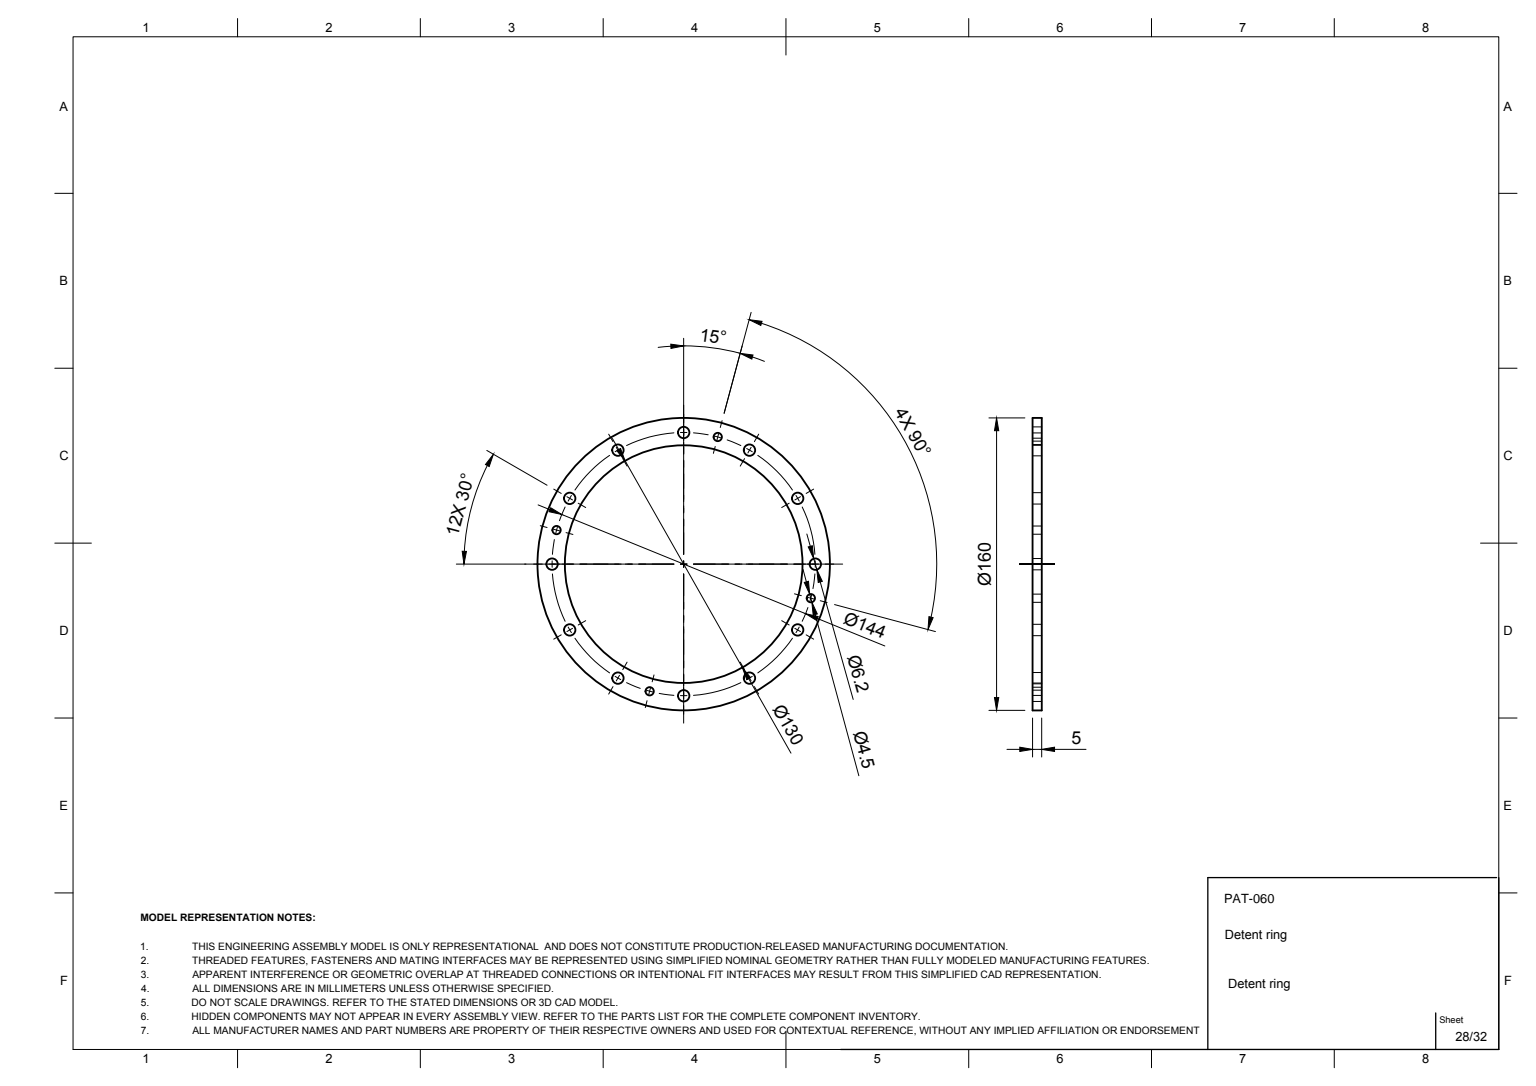
ISO-10303-21;
HEADER;
/* Generated by software containing ST-Developer
 * from STEP Tools, Inc. (www.steptools.com) 
 */

FILE_DESCRIPTION(
/* description */ ('Indexing fixture plate with plunger'),
/* implementation_level */ '2;1');

FILE_NAME(
/* name */ 'Detent ring.step',
/* time_stamp */ '2026-10-28T03:23:41-07:00',
/* author */ (''),
/* organization */ (''),
/* preprocessor_version */ 'ST-DEVELOPER v20.2',
/* originating_system */ 'Autodesk Translation Framework v15.17.0.0',
/* authorisation */ '');

FILE_SCHEMA (('AUTOMOTIVE_DESIGN { 1 0 10303 214 3 1 1 }'));
ENDSEC;

DATA;
#10=MECHANICAL_DESIGN_GEOMETRIC_PRESENTATION_REPRESENTATION('',(#348),#10020);
#285=SHAPE_REPRESENTATION_RELATIONSHIP('SRR','None',#10161,#312);
#312=ADVANCED_BREP_SHAPE_REPRESENTATION('',(#383),#10014);
#348=STYLED_ITEM('',(#10354),#383);
#383=MANIFOLD_SOLID_BREP('Body1',#4603);
#495=FACE_BOUND('',#1306,.T.);
#496=FACE_BOUND('',#1307,.T.);
#497=FACE_BOUND('',#1308,.T.);
#498=FACE_BOUND('',#1309,.T.);
#499=FACE_BOUND('',#1310,.T.);
#500=FACE_BOUND('',#1311,.T.);
#501=FACE_BOUND('',#1312,.T.);
#502=FACE_BOUND('',#1313,.T.);
#503=FACE_BOUND('',#1314,.T.);
#504=FACE_BOUND('',#1315,.T.);
#505=FACE_BOUND('',#1316,.T.);
#506=FACE_BOUND('',#1317,.T.);
#507=FACE_BOUND('',#1318,.T.);
#508=FACE_BOUND('',#1319,.T.);
#509=FACE_BOUND('',#1320,.T.);
#510=FACE_BOUND('',#1321,.T.);
#511=FACE_BOUND('',#1322,.T.);
#512=FACE_BOUND('',#1324,.T.);
#513=FACE_BOUND('',#1325,.T.);
#514=FACE_BOUND('',#1326,.T.);
#515=FACE_BOUND('',#1327,.T.);
#516=FACE_BOUND('',#1328,.T.);
#517=FACE_BOUND('',#1329,.T.);
#518=FACE_BOUND('',#1330,.T.);
#519=FACE_BOUND('',#1331,.T.);
#520=FACE_BOUND('',#1332,.T.);
#521=FACE_BOUND('',#1333,.T.);
#522=FACE_BOUND('',#1334,.T.);
#523=FACE_BOUND('',#1335,.T.);
#524=FACE_BOUND('',#1336,.T.);
#525=FACE_BOUND('',#1337,.T.);
#526=FACE_BOUND('',#1338,.T.);
#527=FACE_BOUND('',#1339,.T.);
#528=FACE_BOUND('',#1340,.T.);
#640=PLANE('',#5458);
#641=PLANE('',#5459);
#893=FACE_OUTER_BOUND('',#1287,.T.);
#894=FACE_OUTER_BOUND('',#1288,.T.);
#895=FACE_OUTER_BOUND('',#1289,.T.);
#896=FACE_OUTER_BOUND('',#1290,.T.);
#897=FACE_OUTER_BOUND('',#1291,.T.);
#898=FACE_OUTER_BOUND('',#1292,.T.);
#899=FACE_OUTER_BOUND('',#1293,.T.);
#900=FACE_OUTER_BOUND('',#1294,.T.);
#901=FACE_OUTER_BOUND('',#1295,.T.);
#902=FACE_OUTER_BOUND('',#1296,.T.);
#903=FACE_OUTER_BOUND('',#1297,.T.);
#904=FACE_OUTER_BOUND('',#1298,.T.);
#905=FACE_OUTER_BOUND('',#1299,.T.);
#906=FACE_OUTER_BOUND('',#1300,.T.);
#907=FACE_OUTER_BOUND('',#1301,.T.);
#908=FACE_OUTER_BOUND('',#1302,.T.);
#909=FACE_OUTER_BOUND('',#1303,.T.);
#910=FACE_OUTER_BOUND('',#1304,.T.);
#911=FACE_OUTER_BOUND('',#1305,.T.);
#912=FACE_OUTER_BOUND('',#1323,.T.);
#1287=EDGE_LOOP('',(#3895,#3896,#3897,#3898));
#1288=EDGE_LOOP('',(#3899,#3900,#3901,#3902));
#1289=EDGE_LOOP('',(#3903,#3904,#3905,#3906));
#1290=EDGE_LOOP('',(#3907,#3908,#3909,#3910));
#1291=EDGE_LOOP('',(#3911,#3912,#3913,#3914));
#1292=EDGE_LOOP('',(#3915,#3916,#3917,#3918));
#1293=EDGE_LOOP('',(#3919,#3920,#3921,#3922));
#1294=EDGE_LOOP('',(#3923,#3924,#3925,#3926));
#1295=EDGE_LOOP('',(#3927,#3928,#3929,#3930));
#1296=EDGE_LOOP('',(#3931,#3932,#3933,#3934));
#1297=EDGE_LOOP('',(#3935,#3936,#3937,#3938));
#1298=EDGE_LOOP('',(#3939,#3940,#3941,#3942));
#1299=EDGE_LOOP('',(#3943,#3944,#3945,#3946));
#1300=EDGE_LOOP('',(#3947,#3948,#3949,#3950));
#1301=EDGE_LOOP('',(#3951,#3952,#3953,#3954));
#1302=EDGE_LOOP('',(#3955,#3956,#3957,#3958));
#1303=EDGE_LOOP('',(#3959,#3960,#3961,#3962));
#1304=EDGE_LOOP('',(#3963,#3964,#3965,#3966));
#1305=EDGE_LOOP('',(#3967));
#1306=EDGE_LOOP('',(#3968));
#1307=EDGE_LOOP('',(#3969));
#1308=EDGE_LOOP('',(#3970));
#1309=EDGE_LOOP('',(#3971));
#1310=EDGE_LOOP('',(#3972));
#1311=EDGE_LOOP('',(#3973));
#1312=EDGE_LOOP('',(#3974));
#1313=EDGE_LOOP('',(#3975));
#1314=EDGE_LOOP('',(#3976));
#1315=EDGE_LOOP('',(#3977));
#1316=EDGE_LOOP('',(#3978));
#1317=EDGE_LOOP('',(#3979));
#1318=EDGE_LOOP('',(#3980));
#1319=EDGE_LOOP('',(#3981));
#1320=EDGE_LOOP('',(#3982));
#1321=EDGE_LOOP('',(#3983));
#1322=EDGE_LOOP('',(#3984));
#1323=EDGE_LOOP('',(#3985));
#1324=EDGE_LOOP('',(#3986));
#1325=EDGE_LOOP('',(#3987));
#1326=EDGE_LOOP('',(#3988));
#1327=EDGE_LOOP('',(#3989));
#1328=EDGE_LOOP('',(#3990));
#1329=EDGE_LOOP('',(#3991));
#1330=EDGE_LOOP('',(#3992));
#1331=EDGE_LOOP('',(#3993));
#1332=EDGE_LOOP('',(#3994));
#1333=EDGE_LOOP('',(#3995));
#1334=EDGE_LOOP('',(#3996));
#1335=EDGE_LOOP('',(#3997));
#1336=EDGE_LOOP('',(#3998));
#1337=EDGE_LOOP('',(#3999));
#1338=EDGE_LOOP('',(#4000));
#1339=EDGE_LOOP('',(#4001));
#1340=EDGE_LOOP('',(#4002));
#1541=LINE('',#9580,#1761);
#1542=LINE('',#9586,#1762);
#1543=LINE('',#9592,#1763);
#1544=LINE('',#9598,#1764);
#1545=LINE('',#9604,#1765);
#1546=LINE('',#9610,#1766);
#1547=LINE('',#9616,#1767);
#1548=LINE('',#9622,#1768);
#1549=LINE('',#9628,#1769);
#1550=LINE('',#9634,#1770);
#1551=LINE('',#9640,#1771);
#1552=LINE('',#9646,#1772);
#1553=LINE('',#9652,#1773);
#1554=LINE('',#9658,#1774);
#1555=LINE('',#9664,#1775);
#1556=LINE('',#9670,#1776);
#1557=LINE('',#9676,#1777);
#1558=LINE('',#9682,#1778);
#1761=VECTOR('',#6720,0.225);
#1762=VECTOR('',#6727,0.225);
#1763=VECTOR('',#6734,0.225);
#1764=VECTOR('',#6741,0.225);
#1765=VECTOR('',#6748,0.31);
#1766=VECTOR('',#6755,0.31);
#1767=VECTOR('',#6762,0.31);
#1768=VECTOR('',#6769,0.31);
#1769=VECTOR('',#6776,0.31);
#1770=VECTOR('',#6783,0.31);
#1771=VECTOR('',#6790,0.31);
#1772=VECTOR('',#6797,0.31);
#1773=VECTOR('',#6804,0.31);
#1774=VECTOR('',#6811,0.31);
#1775=VECTOR('',#6818,0.31);
#1776=VECTOR('',#6825,0.31);
#1777=VECTOR('',#6832,6.5);
#1778=VECTOR('',#6839,8.);
#2075=CIRCLE('',#5405,0.225);
#2076=CIRCLE('',#5406,0.225);
#2077=CIRCLE('',#5408,0.225);
#2078=CIRCLE('',#5409,0.225);
#2079=CIRCLE('',#5411,0.225);
#2080=CIRCLE('',#5412,0.225);
#2081=CIRCLE('',#5414,0.225);
#2082=CIRCLE('',#5415,0.225);
#2083=CIRCLE('',#5417,0.31);
#2084=CIRCLE('',#5418,0.31);
#2085=CIRCLE('',#5420,0.31);
#2086=CIRCLE('',#5421,0.31);
#2087=CIRCLE('',#5423,0.31);
#2088=CIRCLE('',#5424,0.31);
#2089=CIRCLE('',#5426,0.31);
#2090=CIRCLE('',#5427,0.31);
#2091=CIRCLE('',#5429,0.31);
#2092=CIRCLE('',#5430,0.31);
#2093=CIRCLE('',#5432,0.31);
#2094=CIRCLE('',#5433,0.31);
#2095=CIRCLE('',#5435,0.31);
#2096=CIRCLE('',#5436,0.31);
#2097=CIRCLE('',#5438,0.31);
#2098=CIRCLE('',#5439,0.31);
#2099=CIRCLE('',#5441,0.31);
#2100=CIRCLE('',#5442,0.31);
#2101=CIRCLE('',#5444,0.31);
#2102=CIRCLE('',#5445,0.31);
#2103=CIRCLE('',#5447,0.31);
#2104=CIRCLE('',#5448,0.31);
#2105=CIRCLE('',#5450,0.31);
#2106=CIRCLE('',#5451,0.31);
#2107=CIRCLE('',#5453,6.5);
#2108=CIRCLE('',#5454,6.5);
#2109=CIRCLE('',#5456,8.);
#2110=CIRCLE('',#5457,8.);
#2422=VERTEX_POINT('',#9577);
#2423=VERTEX_POINT('',#9579);
#2424=VERTEX_POINT('',#9583);
#2425=VERTEX_POINT('',#9585);
#2426=VERTEX_POINT('',#9589);
#2427=VERTEX_POINT('',#9591);
#2428=VERTEX_POINT('',#9595);
#2429=VERTEX_POINT('',#9597);
#2430=VERTEX_POINT('',#9601);
#2431=VERTEX_POINT('',#9603);
#2432=VERTEX_POINT('',#9607);
#2433=VERTEX_POINT('',#9609);
#2434=VERTEX_POINT('',#9613);
#2435=VERTEX_POINT('',#9615);
#2436=VERTEX_POINT('',#9619);
#2437=VERTEX_POINT('',#9621);
#2438=VERTEX_POINT('',#9625);
#2439=VERTEX_POINT('',#9627);
#2440=VERTEX_POINT('',#9631);
#2441=VERTEX_POINT('',#9633);
#2442=VERTEX_POINT('',#9637);
#2443=VERTEX_POINT('',#9639);
#2444=VERTEX_POINT('',#9643);
#2445=VERTEX_POINT('',#9645);
#2446=VERTEX_POINT('',#9649);
#2447=VERTEX_POINT('',#9651);
#2448=VERTEX_POINT('',#9655);
#2449=VERTEX_POINT('',#9657);
#2450=VERTEX_POINT('',#9661);
#2451=VERTEX_POINT('',#9663);
#2452=VERTEX_POINT('',#9667);
#2453=VERTEX_POINT('',#9669);
#2454=VERTEX_POINT('',#9673);
#2455=VERTEX_POINT('',#9675);
#2456=VERTEX_POINT('',#9679);
#2457=VERTEX_POINT('',#9681);
#2927=EDGE_CURVE('',#2422,#2422,#2075,.T.);
#2928=EDGE_CURVE('',#2422,#2423,#1541,.T.);
#2929=EDGE_CURVE('',#2423,#2423,#2076,.T.);
#2930=EDGE_CURVE('',#2424,#2424,#2077,.T.);
#2931=EDGE_CURVE('',#2424,#2425,#1542,.T.);
#2932=EDGE_CURVE('',#2425,#2425,#2078,.T.);
#2933=EDGE_CURVE('',#2426,#2426,#2079,.T.);
#2934=EDGE_CURVE('',#2426,#2427,#1543,.T.);
#2935=EDGE_CURVE('',#2427,#2427,#2080,.T.);
#2936=EDGE_CURVE('',#2428,#2428,#2081,.T.);
#2937=EDGE_CURVE('',#2428,#2429,#1544,.T.);
#2938=EDGE_CURVE('',#2429,#2429,#2082,.T.);
#2939=EDGE_CURVE('',#2430,#2430,#2083,.T.);
#2940=EDGE_CURVE('',#2430,#2431,#1545,.T.);
#2941=EDGE_CURVE('',#2431,#2431,#2084,.T.);
#2942=EDGE_CURVE('',#2432,#2432,#2085,.T.);
#2943=EDGE_CURVE('',#2432,#2433,#1546,.T.);
#2944=EDGE_CURVE('',#2433,#2433,#2086,.T.);
#2945=EDGE_CURVE('',#2434,#2434,#2087,.T.);
#2946=EDGE_CURVE('',#2434,#2435,#1547,.T.);
#2947=EDGE_CURVE('',#2435,#2435,#2088,.T.);
#2948=EDGE_CURVE('',#2436,#2436,#2089,.T.);
#2949=EDGE_CURVE('',#2436,#2437,#1548,.T.);
#2950=EDGE_CURVE('',#2437,#2437,#2090,.T.);
#2951=EDGE_CURVE('',#2438,#2438,#2091,.T.);
#2952=EDGE_CURVE('',#2438,#2439,#1549,.T.);
#2953=EDGE_CURVE('',#2439,#2439,#2092,.T.);
#2954=EDGE_CURVE('',#2440,#2440,#2093,.T.);
#2955=EDGE_CURVE('',#2440,#2441,#1550,.T.);
#2956=EDGE_CURVE('',#2441,#2441,#2094,.T.);
#2957=EDGE_CURVE('',#2442,#2442,#2095,.T.);
#2958=EDGE_CURVE('',#2442,#2443,#1551,.T.);
#2959=EDGE_CURVE('',#2443,#2443,#2096,.T.);
#2960=EDGE_CURVE('',#2444,#2444,#2097,.T.);
#2961=EDGE_CURVE('',#2444,#2445,#1552,.T.);
#2962=EDGE_CURVE('',#2445,#2445,#2098,.T.);
#2963=EDGE_CURVE('',#2446,#2446,#2099,.T.);
#2964=EDGE_CURVE('',#2446,#2447,#1553,.T.);
#2965=EDGE_CURVE('',#2447,#2447,#2100,.T.);
#2966=EDGE_CURVE('',#2448,#2448,#2101,.T.);
#2967=EDGE_CURVE('',#2448,#2449,#1554,.T.);
#2968=EDGE_CURVE('',#2449,#2449,#2102,.T.);
#2969=EDGE_CURVE('',#2450,#2450,#2103,.T.);
#2970=EDGE_CURVE('',#2450,#2451,#1555,.T.);
#2971=EDGE_CURVE('',#2451,#2451,#2104,.T.);
#2972=EDGE_CURVE('',#2452,#2452,#2105,.T.);
#2973=EDGE_CURVE('',#2452,#2453,#1556,.T.);
#2974=EDGE_CURVE('',#2453,#2453,#2106,.T.);
#2975=EDGE_CURVE('',#2454,#2454,#2107,.T.);
#2976=EDGE_CURVE('',#2454,#2455,#1557,.T.);
#2977=EDGE_CURVE('',#2455,#2455,#2108,.T.);
#2978=EDGE_CURVE('',#2456,#2456,#2109,.T.);
#2979=EDGE_CURVE('',#2456,#2457,#1558,.T.);
#2980=EDGE_CURVE('',#2457,#2457,#2110,.T.);
#3895=ORIENTED_EDGE('',*,*,#2927,.F.);
#3896=ORIENTED_EDGE('',*,*,#2928,.T.);
#3897=ORIENTED_EDGE('',*,*,#2929,.F.);
#3898=ORIENTED_EDGE('',*,*,#2928,.F.);
#3899=ORIENTED_EDGE('',*,*,#2930,.F.);
#3900=ORIENTED_EDGE('',*,*,#2931,.T.);
#3901=ORIENTED_EDGE('',*,*,#2932,.F.);
#3902=ORIENTED_EDGE('',*,*,#2931,.F.);
#3903=ORIENTED_EDGE('',*,*,#2933,.F.);
#3904=ORIENTED_EDGE('',*,*,#2934,.T.);
#3905=ORIENTED_EDGE('',*,*,#2935,.F.);
#3906=ORIENTED_EDGE('',*,*,#2934,.F.);
#3907=ORIENTED_EDGE('',*,*,#2936,.F.);
#3908=ORIENTED_EDGE('',*,*,#2937,.T.);
#3909=ORIENTED_EDGE('',*,*,#2938,.F.);
#3910=ORIENTED_EDGE('',*,*,#2937,.F.);
#3911=ORIENTED_EDGE('',*,*,#2939,.F.);
#3912=ORIENTED_EDGE('',*,*,#2940,.T.);
#3913=ORIENTED_EDGE('',*,*,#2941,.F.);
#3914=ORIENTED_EDGE('',*,*,#2940,.F.);
#3915=ORIENTED_EDGE('',*,*,#2942,.F.);
#3916=ORIENTED_EDGE('',*,*,#2943,.T.);
#3917=ORIENTED_EDGE('',*,*,#2944,.F.);
#3918=ORIENTED_EDGE('',*,*,#2943,.F.);
#3919=ORIENTED_EDGE('',*,*,#2945,.F.);
#3920=ORIENTED_EDGE('',*,*,#2946,.T.);
#3921=ORIENTED_EDGE('',*,*,#2947,.F.);
#3922=ORIENTED_EDGE('',*,*,#2946,.F.);
#3923=ORIENTED_EDGE('',*,*,#2948,.F.);
#3924=ORIENTED_EDGE('',*,*,#2949,.T.);
#3925=ORIENTED_EDGE('',*,*,#2950,.F.);
#3926=ORIENTED_EDGE('',*,*,#2949,.F.);
#3927=ORIENTED_EDGE('',*,*,#2951,.F.);
#3928=ORIENTED_EDGE('',*,*,#2952,.T.);
#3929=ORIENTED_EDGE('',*,*,#2953,.F.);
#3930=ORIENTED_EDGE('',*,*,#2952,.F.);
#3931=ORIENTED_EDGE('',*,*,#2954,.F.);
#3932=ORIENTED_EDGE('',*,*,#2955,.T.);
#3933=ORIENTED_EDGE('',*,*,#2956,.F.);
#3934=ORIENTED_EDGE('',*,*,#2955,.F.);
#3935=ORIENTED_EDGE('',*,*,#2957,.F.);
#3936=ORIENTED_EDGE('',*,*,#2958,.T.);
#3937=ORIENTED_EDGE('',*,*,#2959,.F.);
#3938=ORIENTED_EDGE('',*,*,#2958,.F.);
#3939=ORIENTED_EDGE('',*,*,#2960,.F.);
#3940=ORIENTED_EDGE('',*,*,#2961,.T.);
#3941=ORIENTED_EDGE('',*,*,#2962,.F.);
#3942=ORIENTED_EDGE('',*,*,#2961,.F.);
#3943=ORIENTED_EDGE('',*,*,#2963,.F.);
#3944=ORIENTED_EDGE('',*,*,#2964,.T.);
#3945=ORIENTED_EDGE('',*,*,#2965,.F.);
#3946=ORIENTED_EDGE('',*,*,#2964,.F.);
#3947=ORIENTED_EDGE('',*,*,#2966,.F.);
#3948=ORIENTED_EDGE('',*,*,#2967,.T.);
#3949=ORIENTED_EDGE('',*,*,#2968,.F.);
#3950=ORIENTED_EDGE('',*,*,#2967,.F.);
#3951=ORIENTED_EDGE('',*,*,#2969,.F.);
#3952=ORIENTED_EDGE('',*,*,#2970,.T.);
#3953=ORIENTED_EDGE('',*,*,#2971,.F.);
#3954=ORIENTED_EDGE('',*,*,#2970,.F.);
#3955=ORIENTED_EDGE('',*,*,#2972,.F.);
#3956=ORIENTED_EDGE('',*,*,#2973,.T.);
#3957=ORIENTED_EDGE('',*,*,#2974,.F.);
#3958=ORIENTED_EDGE('',*,*,#2973,.F.);
#3959=ORIENTED_EDGE('',*,*,#2975,.F.);
#3960=ORIENTED_EDGE('',*,*,#2976,.T.);
#3961=ORIENTED_EDGE('',*,*,#2977,.T.);
#3962=ORIENTED_EDGE('',*,*,#2976,.F.);
#3963=ORIENTED_EDGE('',*,*,#2978,.F.);
#3964=ORIENTED_EDGE('',*,*,#2979,.T.);
#3965=ORIENTED_EDGE('',*,*,#2980,.T.);
#3966=ORIENTED_EDGE('',*,*,#2979,.F.);
#3967=ORIENTED_EDGE('',*,*,#2978,.T.);
#3968=ORIENTED_EDGE('',*,*,#2941,.T.);
#3969=ORIENTED_EDGE('',*,*,#2944,.T.);
#3970=ORIENTED_EDGE('',*,*,#2947,.T.);
#3971=ORIENTED_EDGE('',*,*,#2950,.T.);
#3972=ORIENTED_EDGE('',*,*,#2953,.T.);
#3973=ORIENTED_EDGE('',*,*,#2956,.T.);
#3974=ORIENTED_EDGE('',*,*,#2959,.T.);
#3975=ORIENTED_EDGE('',*,*,#2962,.T.);
#3976=ORIENTED_EDGE('',*,*,#2965,.T.);
#3977=ORIENTED_EDGE('',*,*,#2968,.T.);
#3978=ORIENTED_EDGE('',*,*,#2971,.T.);
#3979=ORIENTED_EDGE('',*,*,#2974,.T.);
#3980=ORIENTED_EDGE('',*,*,#2975,.T.);
#3981=ORIENTED_EDGE('',*,*,#2938,.T.);
#3982=ORIENTED_EDGE('',*,*,#2935,.T.);
#3983=ORIENTED_EDGE('',*,*,#2932,.T.);
#3984=ORIENTED_EDGE('',*,*,#2929,.T.);
#3985=ORIENTED_EDGE('',*,*,#2980,.F.);
#3986=ORIENTED_EDGE('',*,*,#2939,.T.);
#3987=ORIENTED_EDGE('',*,*,#2942,.T.);
#3988=ORIENTED_EDGE('',*,*,#2945,.T.);
#3989=ORIENTED_EDGE('',*,*,#2948,.T.);
#3990=ORIENTED_EDGE('',*,*,#2951,.T.);
#3991=ORIENTED_EDGE('',*,*,#2954,.T.);
#3992=ORIENTED_EDGE('',*,*,#2957,.T.);
#3993=ORIENTED_EDGE('',*,*,#2960,.T.);
#3994=ORIENTED_EDGE('',*,*,#2963,.T.);
#3995=ORIENTED_EDGE('',*,*,#2966,.T.);
#3996=ORIENTED_EDGE('',*,*,#2969,.T.);
#3997=ORIENTED_EDGE('',*,*,#2972,.T.);
#3998=ORIENTED_EDGE('',*,*,#2977,.F.);
#3999=ORIENTED_EDGE('',*,*,#2936,.T.);
#4000=ORIENTED_EDGE('',*,*,#2933,.T.);
#4001=ORIENTED_EDGE('',*,*,#2930,.T.);
#4002=ORIENTED_EDGE('',*,*,#2927,.T.);
#4258=CYLINDRICAL_SURFACE('',#5404,0.225);
#4259=CYLINDRICAL_SURFACE('',#5407,0.225);
#4260=CYLINDRICAL_SURFACE('',#5410,0.225);
#4261=CYLINDRICAL_SURFACE('',#5413,0.225);
#4262=CYLINDRICAL_SURFACE('',#5416,0.31);
#4263=CYLINDRICAL_SURFACE('',#5419,0.31);
#4264=CYLINDRICAL_SURFACE('',#5422,0.31);
#4265=CYLINDRICAL_SURFACE('',#5425,0.31);
#4266=CYLINDRICAL_SURFACE('',#5428,0.31);
#4267=CYLINDRICAL_SURFACE('',#5431,0.31);
#4268=CYLINDRICAL_SURFACE('',#5434,0.31);
#4269=CYLINDRICAL_SURFACE('',#5437,0.31);
#4270=CYLINDRICAL_SURFACE('',#5440,0.31);
#4271=CYLINDRICAL_SURFACE('',#5443,0.31);
#4272=CYLINDRICAL_SURFACE('',#5446,0.31);
#4273=CYLINDRICAL_SURFACE('',#5449,0.31);
#4274=CYLINDRICAL_SURFACE('',#5452,6.5);
#4275=CYLINDRICAL_SURFACE('',#5455,8.);
#4508=ADVANCED_FACE('',(#893),#4258,.F.);
#4509=ADVANCED_FACE('',(#894),#4259,.F.);
#4510=ADVANCED_FACE('',(#895),#4260,.F.);
#4511=ADVANCED_FACE('',(#896),#4261,.F.);
#4512=ADVANCED_FACE('',(#897),#4262,.F.);
#4513=ADVANCED_FACE('',(#898),#4263,.F.);
#4514=ADVANCED_FACE('',(#899),#4264,.F.);
#4515=ADVANCED_FACE('',(#900),#4265,.F.);
#4516=ADVANCED_FACE('',(#901),#4266,.F.);
#4517=ADVANCED_FACE('',(#902),#4267,.F.);
#4518=ADVANCED_FACE('',(#903),#4268,.F.);
#4519=ADVANCED_FACE('',(#904),#4269,.F.);
#4520=ADVANCED_FACE('',(#905),#4270,.F.);
#4521=ADVANCED_FACE('',(#906),#4271,.F.);
#4522=ADVANCED_FACE('',(#907),#4272,.F.);
#4523=ADVANCED_FACE('',(#908),#4273,.F.);
#4524=ADVANCED_FACE('',(#909),#4274,.F.);
#4525=ADVANCED_FACE('',(#910),#4275,.T.);
#4526=ADVANCED_FACE('',(#911,#495,#496,#497,#498,#499,#500,#501,#502,#503,
#504,#505,#506,#507,#508,#509,#510,#511),#640,.T.);
#4527=ADVANCED_FACE('',(#912,#512,#513,#514,#515,#516,#517,#518,#519,#520,
#521,#522,#523,#524,#525,#526,#527,#528),#641,.F.);
#4603=CLOSED_SHELL('',(#4508,#4509,#4510,#4511,#4512,#4513,#4514,#4515,
#4516,#4517,#4518,#4519,#4520,#4521,#4522,#4523,#4524,#4525,#4526,#4527));
#5403=AXIS2_PLACEMENT_3D('',#9575,#6714,#6715);
#5404=AXIS2_PLACEMENT_3D('',#9576,#6716,#6717);
#5405=AXIS2_PLACEMENT_3D('',#9578,#6718,#6719);
#5406=AXIS2_PLACEMENT_3D('',#9581,#6721,#6722);
#5407=AXIS2_PLACEMENT_3D('',#9582,#6723,#6724);
#5408=AXIS2_PLACEMENT_3D('',#9584,#6725,#6726);
#5409=AXIS2_PLACEMENT_3D('',#9587,#6728,#6729);
#5410=AXIS2_PLACEMENT_3D('',#9588,#6730,#6731);
#5411=AXIS2_PLACEMENT_3D('',#9590,#6732,#6733);
#5412=AXIS2_PLACEMENT_3D('',#9593,#6735,#6736);
#5413=AXIS2_PLACEMENT_3D('',#9594,#6737,#6738);
#5414=AXIS2_PLACEMENT_3D('',#9596,#6739,#6740);
#5415=AXIS2_PLACEMENT_3D('',#9599,#6742,#6743);
#5416=AXIS2_PLACEMENT_3D('',#9600,#6744,#6745);
#5417=AXIS2_PLACEMENT_3D('',#9602,#6746,#6747);
#5418=AXIS2_PLACEMENT_3D('',#9605,#6749,#6750);
#5419=AXIS2_PLACEMENT_3D('',#9606,#6751,#6752);
#5420=AXIS2_PLACEMENT_3D('',#9608,#6753,#6754);
#5421=AXIS2_PLACEMENT_3D('',#9611,#6756,#6757);
#5422=AXIS2_PLACEMENT_3D('',#9612,#6758,#6759);
#5423=AXIS2_PLACEMENT_3D('',#9614,#6760,#6761);
#5424=AXIS2_PLACEMENT_3D('',#9617,#6763,#6764);
#5425=AXIS2_PLACEMENT_3D('',#9618,#6765,#6766);
#5426=AXIS2_PLACEMENT_3D('',#9620,#6767,#6768);
#5427=AXIS2_PLACEMENT_3D('',#9623,#6770,#6771);
#5428=AXIS2_PLACEMENT_3D('',#9624,#6772,#6773);
#5429=AXIS2_PLACEMENT_3D('',#9626,#6774,#6775);
#5430=AXIS2_PLACEMENT_3D('',#9629,#6777,#6778);
#5431=AXIS2_PLACEMENT_3D('',#9630,#6779,#6780);
#5432=AXIS2_PLACEMENT_3D('',#9632,#6781,#6782);
#5433=AXIS2_PLACEMENT_3D('',#9635,#6784,#6785);
#5434=AXIS2_PLACEMENT_3D('',#9636,#6786,#6787);
#5435=AXIS2_PLACEMENT_3D('',#9638,#6788,#6789);
#5436=AXIS2_PLACEMENT_3D('',#9641,#6791,#6792);
#5437=AXIS2_PLACEMENT_3D('',#9642,#6793,#6794);
#5438=AXIS2_PLACEMENT_3D('',#9644,#6795,#6796);
#5439=AXIS2_PLACEMENT_3D('',#9647,#6798,#6799);
#5440=AXIS2_PLACEMENT_3D('',#9648,#6800,#6801);
#5441=AXIS2_PLACEMENT_3D('',#9650,#6802,#6803);
#5442=AXIS2_PLACEMENT_3D('',#9653,#6805,#6806);
#5443=AXIS2_PLACEMENT_3D('',#9654,#6807,#6808);
#5444=AXIS2_PLACEMENT_3D('',#9656,#6809,#6810);
#5445=AXIS2_PLACEMENT_3D('',#9659,#6812,#6813);
#5446=AXIS2_PLACEMENT_3D('',#9660,#6814,#6815);
#5447=AXIS2_PLACEMENT_3D('',#9662,#6816,#6817);
#5448=AXIS2_PLACEMENT_3D('',#9665,#6819,#6820);
#5449=AXIS2_PLACEMENT_3D('',#9666,#6821,#6822);
#5450=AXIS2_PLACEMENT_3D('',#9668,#6823,#6824);
#5451=AXIS2_PLACEMENT_3D('',#9671,#6826,#6827);
#5452=AXIS2_PLACEMENT_3D('',#9672,#6828,#6829);
#5453=AXIS2_PLACEMENT_3D('',#9674,#6830,#6831);
#5454=AXIS2_PLACEMENT_3D('',#9677,#6833,#6834);
#5455=AXIS2_PLACEMENT_3D('',#9678,#6835,#6836);
#5456=AXIS2_PLACEMENT_3D('',#9680,#6837,#6838);
#5457=AXIS2_PLACEMENT_3D('',#9683,#6840,#6841);
#5458=AXIS2_PLACEMENT_3D('',#9684,#6842,#6843);
#5459=AXIS2_PLACEMENT_3D('',#9685,#6844,#6845);
#6714=DIRECTION('axis',(0.,0.,1.));
#6715=DIRECTION('refdir',(1.,0.,0.));
#6716=DIRECTION('center_axis',(0.,0.,1.));
#6717=DIRECTION('ref_axis',(1.,0.,0.));
#6718=DIRECTION('center_axis',(0.,0.,1.));
#6719=DIRECTION('ref_axis',(1.,0.,0.));
#6720=DIRECTION('',(0.,0.,1.));
#6721=DIRECTION('center_axis',(0.,0.,-1.));
#6722=DIRECTION('ref_axis',(1.,0.,0.));
#6723=DIRECTION('center_axis',(0.,0.,1.));
#6724=DIRECTION('ref_axis',(1.,0.,0.));
#6725=DIRECTION('center_axis',(0.,0.,1.));
#6726=DIRECTION('ref_axis',(1.,0.,0.));
#6727=DIRECTION('',(0.,0.,1.));
#6728=DIRECTION('center_axis',(0.,0.,-1.));
#6729=DIRECTION('ref_axis',(1.,0.,0.));
#6730=DIRECTION('center_axis',(0.,0.,1.));
#6731=DIRECTION('ref_axis',(1.,0.,0.));
#6732=DIRECTION('center_axis',(0.,0.,1.));
#6733=DIRECTION('ref_axis',(1.,0.,0.));
#6734=DIRECTION('',(0.,0.,1.));
#6735=DIRECTION('center_axis',(0.,0.,-1.));
#6736=DIRECTION('ref_axis',(1.,0.,0.));
#6737=DIRECTION('center_axis',(0.,0.,1.));
#6738=DIRECTION('ref_axis',(1.,0.,0.));
#6739=DIRECTION('center_axis',(0.,0.,1.));
#6740=DIRECTION('ref_axis',(1.,0.,0.));
#6741=DIRECTION('',(0.,0.,1.));
#6742=DIRECTION('center_axis',(0.,0.,-1.));
#6743=DIRECTION('ref_axis',(1.,0.,0.));
#6744=DIRECTION('center_axis',(0.,0.,1.));
#6745=DIRECTION('ref_axis',(1.,0.,0.));
#6746=DIRECTION('center_axis',(0.,0.,1.));
#6747=DIRECTION('ref_axis',(1.,0.,0.));
#6748=DIRECTION('',(0.,0.,1.));
#6749=DIRECTION('center_axis',(0.,0.,-1.));
#6750=DIRECTION('ref_axis',(1.,0.,0.));
#6751=DIRECTION('center_axis',(0.,0.,1.));
#6752=DIRECTION('ref_axis',(1.,0.,0.));
#6753=DIRECTION('center_axis',(0.,0.,1.));
#6754=DIRECTION('ref_axis',(1.,0.,0.));
#6755=DIRECTION('',(0.,0.,1.));
#6756=DIRECTION('center_axis',(0.,0.,-1.));
#6757=DIRECTION('ref_axis',(1.,0.,0.));
#6758=DIRECTION('center_axis',(0.,0.,1.));
#6759=DIRECTION('ref_axis',(1.,0.,0.));
#6760=DIRECTION('center_axis',(0.,0.,1.));
#6761=DIRECTION('ref_axis',(1.,0.,0.));
#6762=DIRECTION('',(0.,0.,1.));
#6763=DIRECTION('center_axis',(0.,0.,-1.));
#6764=DIRECTION('ref_axis',(1.,0.,0.));
#6765=DIRECTION('center_axis',(0.,0.,1.));
#6766=DIRECTION('ref_axis',(1.,0.,0.));
#6767=DIRECTION('center_axis',(0.,0.,1.));
#6768=DIRECTION('ref_axis',(1.,0.,0.));
#6769=DIRECTION('',(0.,0.,1.));
#6770=DIRECTION('center_axis',(0.,0.,-1.));
#6771=DIRECTION('ref_axis',(1.,0.,0.));
#6772=DIRECTION('center_axis',(0.,0.,1.));
#6773=DIRECTION('ref_axis',(1.,0.,0.));
#6774=DIRECTION('center_axis',(0.,0.,1.));
#6775=DIRECTION('ref_axis',(1.,0.,0.));
#6776=DIRECTION('',(0.,0.,1.));
#6777=DIRECTION('center_axis',(0.,0.,-1.));
#6778=DIRECTION('ref_axis',(1.,0.,0.));
#6779=DIRECTION('center_axis',(0.,0.,1.));
#6780=DIRECTION('ref_axis',(1.,0.,0.));
#6781=DIRECTION('center_axis',(0.,0.,1.));
#6782=DIRECTION('ref_axis',(1.,0.,0.));
#6783=DIRECTION('',(0.,0.,1.));
#6784=DIRECTION('center_axis',(0.,0.,-1.));
#6785=DIRECTION('ref_axis',(1.,0.,0.));
#6786=DIRECTION('center_axis',(0.,0.,1.));
#6787=DIRECTION('ref_axis',(1.,0.,0.));
#6788=DIRECTION('center_axis',(0.,0.,1.));
#6789=DIRECTION('ref_axis',(1.,0.,0.));
#6790=DIRECTION('',(0.,0.,1.));
#6791=DIRECTION('center_axis',(0.,0.,-1.));
#6792=DIRECTION('ref_axis',(1.,0.,0.));
#6793=DIRECTION('center_axis',(0.,0.,1.));
#6794=DIRECTION('ref_axis',(1.,0.,0.));
#6795=DIRECTION('center_axis',(0.,0.,1.));
#6796=DIRECTION('ref_axis',(1.,0.,0.));
#6797=DIRECTION('',(0.,0.,1.));
#6798=DIRECTION('center_axis',(0.,0.,-1.));
#6799=DIRECTION('ref_axis',(1.,0.,0.));
#6800=DIRECTION('center_axis',(0.,0.,1.));
#6801=DIRECTION('ref_axis',(1.,0.,0.));
#6802=DIRECTION('center_axis',(0.,0.,1.));
#6803=DIRECTION('ref_axis',(1.,0.,0.));
#6804=DIRECTION('',(0.,0.,1.));
#6805=DIRECTION('center_axis',(0.,0.,-1.));
#6806=DIRECTION('ref_axis',(1.,0.,0.));
#6807=DIRECTION('center_axis',(0.,0.,1.));
#6808=DIRECTION('ref_axis',(1.,0.,0.));
#6809=DIRECTION('center_axis',(0.,0.,1.));
#6810=DIRECTION('ref_axis',(1.,0.,0.));
#6811=DIRECTION('',(0.,0.,1.));
#6812=DIRECTION('center_axis',(0.,0.,-1.));
#6813=DIRECTION('ref_axis',(1.,0.,0.));
#6814=DIRECTION('center_axis',(0.,0.,1.));
#6815=DIRECTION('ref_axis',(1.,0.,0.));
#6816=DIRECTION('center_axis',(0.,0.,1.));
#6817=DIRECTION('ref_axis',(1.,0.,0.));
#6818=DIRECTION('',(0.,0.,1.));
#6819=DIRECTION('center_axis',(0.,0.,-1.));
#6820=DIRECTION('ref_axis',(1.,0.,0.));
#6821=DIRECTION('center_axis',(0.,0.,1.));
#6822=DIRECTION('ref_axis',(1.,0.,0.));
#6823=DIRECTION('center_axis',(0.,0.,1.));
#6824=DIRECTION('ref_axis',(1.,0.,0.));
#6825=DIRECTION('',(0.,0.,1.));
#6826=DIRECTION('center_axis',(0.,0.,-1.));
#6827=DIRECTION('ref_axis',(1.,0.,0.));
#6828=DIRECTION('center_axis',(0.,0.,1.));
#6829=DIRECTION('ref_axis',(1.,0.,0.));
#6830=DIRECTION('center_axis',(0.,0.,-1.));
#6831=DIRECTION('ref_axis',(1.,0.,0.));
#6832=DIRECTION('',(0.,0.,-1.));
#6833=DIRECTION('center_axis',(0.,0.,-1.));
#6834=DIRECTION('ref_axis',(1.,0.,0.));
#6835=DIRECTION('center_axis',(0.,0.,1.));
#6836=DIRECTION('ref_axis',(1.,0.,0.));
#6837=DIRECTION('center_axis',(0.,0.,1.));
#6838=DIRECTION('ref_axis',(1.,0.,0.));
#6839=DIRECTION('',(0.,0.,-1.));
#6840=DIRECTION('center_axis',(0.,0.,1.));
#6841=DIRECTION('ref_axis',(1.,0.,0.));
#6842=DIRECTION('center_axis',(0.,0.,1.));
#6843=DIRECTION('ref_axis',(1.,0.,0.));
#6844=DIRECTION('center_axis',(0.,0.,1.));
#6845=DIRECTION('ref_axis',(1.,0.,0.));
#9575=CARTESIAN_POINT('',(0.,0.,0.));
#9576=CARTESIAN_POINT('Origin',(-6.95466594928129,-1.86349712473815,5.9));
#9577=CARTESIAN_POINT('',(-7.17966594928129,-1.86349712473815,6.));
#9578=CARTESIAN_POINT('Origin',(-6.95466594928129,-1.86349712473815,6.));
#9579=CARTESIAN_POINT('',(-7.17966594928129,-1.86349712473815,6.5));
#9580=CARTESIAN_POINT('',(-7.17966594928129,-1.86349712473815,5.9));
#9581=CARTESIAN_POINT('Origin',(-6.95466594928129,-1.86349712473815,6.5));
#9582=CARTESIAN_POINT('Origin',(-1.86349712473815,6.95466594928129,5.9));
#9583=CARTESIAN_POINT('',(-2.08849712473815,6.95466594928129,6.));
#9584=CARTESIAN_POINT('Origin',(-1.86349712473815,6.95466594928129,6.));
#9585=CARTESIAN_POINT('',(-2.08849712473815,6.95466594928129,6.5));
#9586=CARTESIAN_POINT('',(-2.08849712473815,6.95466594928129,5.9));
#9587=CARTESIAN_POINT('Origin',(-1.86349712473815,6.95466594928129,6.5));
#9588=CARTESIAN_POINT('Origin',(6.95466594928129,1.86349712473815,5.9));
#9589=CARTESIAN_POINT('',(6.72966594928129,1.86349712473815,6.));
#9590=CARTESIAN_POINT('Origin',(6.95466594928129,1.86349712473815,6.));
#9591=CARTESIAN_POINT('',(6.72966594928129,1.86349712473815,6.5));
#9592=CARTESIAN_POINT('',(6.72966594928129,1.86349712473815,5.9));
#9593=CARTESIAN_POINT('Origin',(6.95466594928129,1.86349712473815,6.5));
#9594=CARTESIAN_POINT('Origin',(1.86349712473815,-6.95466594928129,5.9));
#9595=CARTESIAN_POINT('',(1.63849712473815,-6.95466594928129,6.));
#9596=CARTESIAN_POINT('Origin',(1.86349712473815,-6.95466594928129,6.));
#9597=CARTESIAN_POINT('',(1.63849712473815,-6.95466594928129,6.5));
#9598=CARTESIAN_POINT('',(1.63849712473815,-6.95466594928129,5.9));
#9599=CARTESIAN_POINT('Origin',(1.86349712473815,-6.95466594928129,6.5));
#9600=CARTESIAN_POINT('Origin',(3.6,-6.23538290724796,5.9));
#9601=CARTESIAN_POINT('',(3.29,-6.23538290724796,6.));
#9602=CARTESIAN_POINT('Origin',(3.6,-6.23538290724796,6.));
#9603=CARTESIAN_POINT('',(3.29,-6.23538290724796,6.5));
#9604=CARTESIAN_POINT('',(3.29,-6.23538290724796,5.9));
#9605=CARTESIAN_POINT('Origin',(3.6,-6.23538290724796,6.5));
#9606=CARTESIAN_POINT('Origin',(-3.6,-6.23538290724796,5.9));
#9607=CARTESIAN_POINT('',(-3.91,-6.23538290724796,6.));
#9608=CARTESIAN_POINT('Origin',(-3.6,-6.23538290724796,6.));
#9609=CARTESIAN_POINT('',(-3.91,-6.23538290724796,6.5));
#9610=CARTESIAN_POINT('',(-3.91,-6.23538290724796,5.9));
#9611=CARTESIAN_POINT('Origin',(-3.6,-6.23538290724796,6.5));
#9612=CARTESIAN_POINT('Origin',(-7.2,8.81745695386094E-16,5.9));
#9613=CARTESIAN_POINT('',(-7.51,8.43781644612526E-16,6.));
#9614=CARTESIAN_POINT('Origin',(-7.2,8.81745695386094E-16,6.));
#9615=CARTESIAN_POINT('',(-7.51,9.19709746159662E-16,6.5));
#9616=CARTESIAN_POINT('',(-7.51,8.43781644612526E-16,5.9));
#9617=CARTESIAN_POINT('Origin',(-7.2,8.81745695386094E-16,6.5));
#9618=CARTESIAN_POINT('Origin',(-6.23538290724796,3.6,5.9));
#9619=CARTESIAN_POINT('',(-6.54538290724796,3.6,6.));
#9620=CARTESIAN_POINT('Origin',(-6.23538290724796,3.6,6.));
#9621=CARTESIAN_POINT('',(-6.54538290724796,3.6,6.5));
#9622=CARTESIAN_POINT('',(-6.54538290724796,3.6,5.9));
#9623=CARTESIAN_POINT('Origin',(-6.23538290724796,3.6,6.5));
#9624=CARTESIAN_POINT('Origin',(4.40872847693047E-16,7.2,5.9));
#9625=CARTESIAN_POINT('',(-0.31,7.2,6.));
#9626=CARTESIAN_POINT('Origin',(4.40872847693047E-16,7.2,6.));
#9627=CARTESIAN_POINT('',(-0.31,7.2,6.5));
#9628=CARTESIAN_POINT('',(-0.31,7.2,5.9));
#9629=CARTESIAN_POINT('Origin',(4.40872847693047E-16,7.2,6.5));
#9630=CARTESIAN_POINT('Origin',(6.23538290724796,3.6,5.9));
#9631=CARTESIAN_POINT('',(5.92538290724796,3.6,6.));
#9632=CARTESIAN_POINT('Origin',(6.23538290724796,3.6,6.));
#9633=CARTESIAN_POINT('',(5.92538290724796,3.6,6.5));
#9634=CARTESIAN_POINT('',(5.92538290724796,3.6,5.9));
#9635=CARTESIAN_POINT('Origin',(6.23538290724796,3.6,6.5));
#9636=CARTESIAN_POINT('Origin',(3.6,6.23538290724796,5.9));
#9637=CARTESIAN_POINT('',(3.29,6.23538290724796,6.));
#9638=CARTESIAN_POINT('Origin',(3.6,6.23538290724796,6.));
#9639=CARTESIAN_POINT('',(3.29,6.23538290724796,6.5));
#9640=CARTESIAN_POINT('',(3.29,6.23538290724796,5.9));
#9641=CARTESIAN_POINT('Origin',(3.6,6.23538290724796,6.5));
#9642=CARTESIAN_POINT('Origin',(-3.6,6.23538290724796,5.9));
#9643=CARTESIAN_POINT('',(-3.91,6.23538290724796,6.));
#9644=CARTESIAN_POINT('Origin',(-3.6,6.23538290724796,6.));
#9645=CARTESIAN_POINT('',(-3.91,6.23538290724796,6.5));
#9646=CARTESIAN_POINT('',(-3.91,6.23538290724796,5.9));
#9647=CARTESIAN_POINT('Origin',(-3.6,6.23538290724796,6.5));
#9648=CARTESIAN_POINT('Origin',(7.2,0.,5.9));
#9649=CARTESIAN_POINT('',(6.89,-3.79640507735679E-17,6.));
#9650=CARTESIAN_POINT('Origin',(7.2,0.,6.));
#9651=CARTESIAN_POINT('',(6.89,3.79640507735679E-17,6.5));
#9652=CARTESIAN_POINT('',(6.89,-3.79640507735679E-17,5.9));
#9653=CARTESIAN_POINT('Origin',(7.2,0.,6.5));
#9654=CARTESIAN_POINT('Origin',(-6.23538290724796,-3.6,5.9));
#9655=CARTESIAN_POINT('',(-6.54538290724796,-3.6,6.));
#9656=CARTESIAN_POINT('Origin',(-6.23538290724796,-3.6,6.));
#9657=CARTESIAN_POINT('',(-6.54538290724796,-3.6,6.5));
#9658=CARTESIAN_POINT('',(-6.54538290724796,-3.6,5.9));
#9659=CARTESIAN_POINT('Origin',(-6.23538290724796,-3.6,6.5));
#9660=CARTESIAN_POINT('Origin',(-1.32261854307914E-15,-7.2,5.9));
#9661=CARTESIAN_POINT('',(-0.310000000000001,-7.2,6.));
#9662=CARTESIAN_POINT('Origin',(-1.32261854307914E-15,-7.2,6.));
#9663=CARTESIAN_POINT('',(-0.310000000000001,-7.2,6.5));
#9664=CARTESIAN_POINT('',(-0.310000000000001,-7.2,5.9));
#9665=CARTESIAN_POINT('Origin',(-1.32261854307914E-15,-7.2,6.5));
#9666=CARTESIAN_POINT('Origin',(6.23538290724796,-3.6,5.9));
#9667=CARTESIAN_POINT('',(5.92538290724796,-3.6,6.));
#9668=CARTESIAN_POINT('Origin',(6.23538290724796,-3.6,6.));
#9669=CARTESIAN_POINT('',(5.92538290724796,-3.6,6.5));
#9670=CARTESIAN_POINT('',(5.92538290724796,-3.6,5.9));
#9671=CARTESIAN_POINT('Origin',(6.23538290724796,-3.6,6.5));
#9672=CARTESIAN_POINT('Origin',(0.,0.,6.));
#9673=CARTESIAN_POINT('',(-6.5,-7.9602041944578E-16,6.5));
#9674=CARTESIAN_POINT('Origin',(0.,0.,6.5));
#9675=CARTESIAN_POINT('',(-6.5,-7.9602041944578E-16,6.));
#9676=CARTESIAN_POINT('',(-6.5,-7.9602041944578E-16,6.));
#9677=CARTESIAN_POINT('Origin',(0.,0.,6.));
#9678=CARTESIAN_POINT('Origin',(0.,0.,6.));
#9679=CARTESIAN_POINT('',(-8.,-9.79717439317883E-16,6.5));
#9680=CARTESIAN_POINT('Origin',(0.,0.,6.5));
#9681=CARTESIAN_POINT('',(-8.,-9.79717439317883E-16,6.));
#9682=CARTESIAN_POINT('',(-8.,-9.79717439317883E-16,6.));
#9683=CARTESIAN_POINT('Origin',(0.,0.,6.));
#9684=CARTESIAN_POINT('Origin',(0.,0.,6.5));
#9685=CARTESIAN_POINT('Origin',(0.,0.,6.));
#9981=UNCERTAINTY_MEASURE_WITH_UNIT(LENGTH_MEASURE(0.001),#10021,
'DISTANCE_ACCURACY_VALUE',
'Maximum model space distance between geometric entities at asserted c
onnectivities');
#9987=UNCERTAINTY_MEASURE_WITH_UNIT(LENGTH_MEASURE(0.001),#10021,
'DISTANCE_ACCURACY_VALUE',
'Maximum model space distance between geometric entities at asserted c
onnectivities');
#10014=(
GEOMETRIC_REPRESENTATION_CONTEXT(3)
GLOBAL_UNCERTAINTY_ASSIGNED_CONTEXT((#9981))
GLOBAL_UNIT_ASSIGNED_CONTEXT((#10021,#10023,#10024))
REPRESENTATION_CONTEXT('','3D')
);
#10020=(
GEOMETRIC_REPRESENTATION_CONTEXT(3)
GLOBAL_UNCERTAINTY_ASSIGNED_CONTEXT((#9987))
GLOBAL_UNIT_ASSIGNED_CONTEXT((#10021,#10023,#10024))
REPRESENTATION_CONTEXT('','3D')
);
#10021=(
LENGTH_UNIT()
NAMED_UNIT(*)
SI_UNIT(.CENTI.,.METRE.)
);
#10023=(
NAMED_UNIT(*)
PLANE_ANGLE_UNIT()
SI_UNIT($,.RADIAN.)
);
#10024=(
NAMED_UNIT(*)
SI_UNIT($,.STERADIAN.)
SOLID_ANGLE_UNIT()
);
#10051=SHAPE_DEFINITION_REPRESENTATION(#10088,#10161);
#10088=PRODUCT_DEFINITION_SHAPE('',$,#10194);
#10161=SHAPE_REPRESENTATION('',(#5403),#10014);
#10167=PRODUCT_DEFINITION_CONTEXT('part definition',#10265,'design');
#10194=PRODUCT_DEFINITION('Detent ring','Detent ring',#10226,#10167);
#10226=PRODUCT_DEFINITION_FORMATION('',$,#10293);
#10265=APPLICATION_CONTEXT(
'Core Data for Automotive Mechanical Design Process');
#10266=PRODUCT_CONTEXT('part definition',#10265,'mechanical');
#10293=PRODUCT('Detent ring','Detent ring','Detent ring',(#10266));
#10348=COLOUR_RGB('Light Blue',0.38,0.62,0.78);
#10349=FILL_AREA_STYLE_COLOUR('',#10348);
#10350=FILL_AREA_STYLE('',(#10349));
#10351=SURFACE_STYLE_FILL_AREA(#10350);
#10352=SURFACE_SIDE_STYLE('',(#10351));
#10353=SURFACE_STYLE_USAGE(.BOTH.,#10352);
#10354=PRESENTATION_STYLE_ASSIGNMENT((#10353));
ENDSEC;
END-ISO-10303-21;
